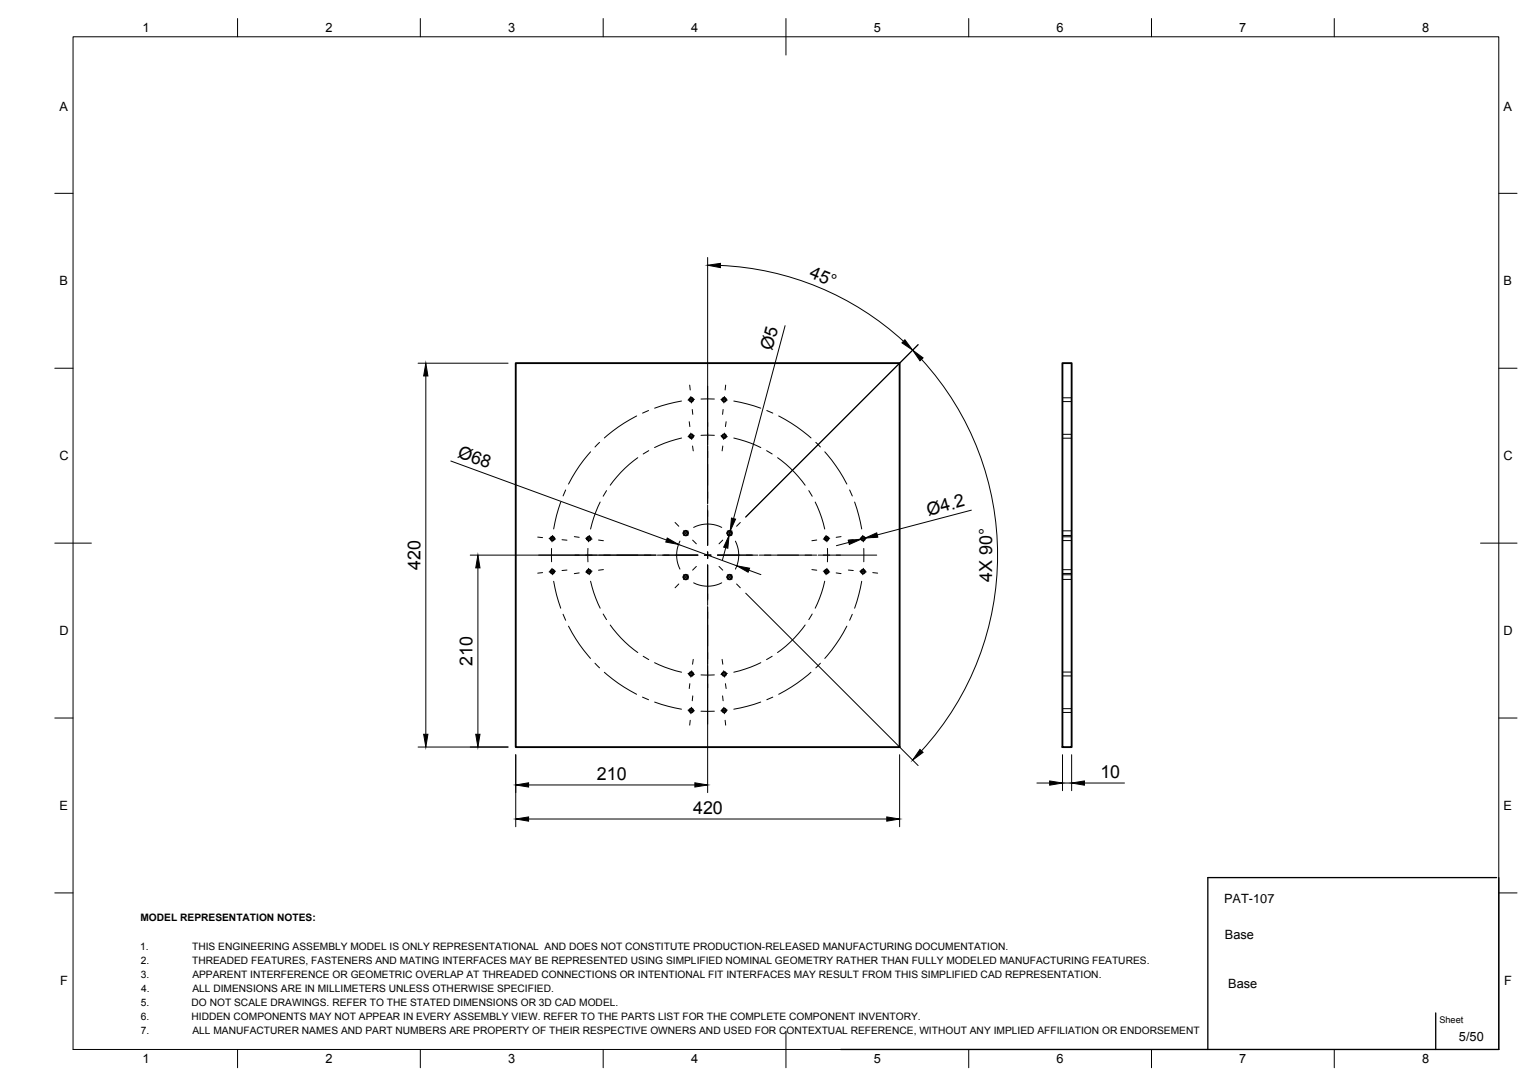
ISO-10303-21;
HEADER;
/* Generated by software containing ST-Developer
 * from STEP Tools, Inc. (www.steptools.com) 
 */

FILE_DESCRIPTION(
/* description */ ('Turntable on roller ring'),
/* implementation_level */ '2;1');

FILE_NAME(
/* name */ 'Base.step',
/* time_stamp */ '2026-10-28T03:23:59-07:00',
/* author */ (''),
/* organization */ (''),
/* preprocessor_version */ 'ST-DEVELOPER v20.2',
/* originating_system */ 'Autodesk Translation Framework v15.17.0.0',
/* authorisation */ '');

FILE_SCHEMA (('AUTOMOTIVE_DESIGN { 1 0 10303 214 3 1 1 }'));
ENDSEC;

DATA;
#10=MECHANICAL_DESIGN_GEOMETRIC_PRESENTATION_REPRESENTATION('',(#617),#16281);
#507=SHAPE_REPRESENTATION_RELATIONSHIP('SRR','None',#16521,#562);
#562=ADVANCED_BREP_SHAPE_REPRESENTATION('',(#689),#16215);
#617=STYLED_ITEM('',(#16911),#689);
#689=MANIFOLD_SOLID_BREP('Body1',#8358);
#757=FACE_BOUND('',#1780,.T.);
#758=FACE_BOUND('',#1781,.T.);
#759=FACE_BOUND('',#1782,.T.);
#760=FACE_BOUND('',#1783,.T.);
#761=FACE_BOUND('',#1784,.T.);
#762=FACE_BOUND('',#1785,.T.);
#763=FACE_BOUND('',#1786,.T.);
#764=FACE_BOUND('',#1787,.T.);
#765=FACE_BOUND('',#1788,.T.);
#766=FACE_BOUND('',#1789,.T.);
#767=FACE_BOUND('',#1790,.T.);
#768=FACE_BOUND('',#1791,.T.);
#769=FACE_BOUND('',#1792,.T.);
#770=FACE_BOUND('',#1793,.T.);
#771=FACE_BOUND('',#1794,.T.);
#772=FACE_BOUND('',#1795,.T.);
#773=FACE_BOUND('',#1796,.T.);
#774=FACE_BOUND('',#1797,.T.);
#775=FACE_BOUND('',#1798,.T.);
#776=FACE_BOUND('',#1799,.T.);
#777=FACE_BOUND('',#1801,.T.);
#778=FACE_BOUND('',#1802,.T.);
#779=FACE_BOUND('',#1803,.T.);
#780=FACE_BOUND('',#1804,.T.);
#781=FACE_BOUND('',#1805,.T.);
#782=FACE_BOUND('',#1806,.T.);
#783=FACE_BOUND('',#1807,.T.);
#784=FACE_BOUND('',#1808,.T.);
#785=FACE_BOUND('',#1809,.T.);
#786=FACE_BOUND('',#1810,.T.);
#787=FACE_BOUND('',#1811,.T.);
#788=FACE_BOUND('',#1812,.T.);
#789=FACE_BOUND('',#1813,.T.);
#790=FACE_BOUND('',#1814,.T.);
#791=FACE_BOUND('',#1815,.T.);
#792=FACE_BOUND('',#1816,.T.);
#793=FACE_BOUND('',#1817,.T.);
#794=FACE_BOUND('',#1818,.T.);
#795=FACE_BOUND('',#1819,.T.);
#796=FACE_BOUND('',#1820,.T.);
#990=PLANE('',#9103);
#991=PLANE('',#9104);
#992=PLANE('',#9105);
#993=PLANE('',#9106);
#994=PLANE('',#9107);
#995=PLANE('',#9108);
#1250=FACE_OUTER_BOUND('',#1755,.T.);
#1251=FACE_OUTER_BOUND('',#1756,.T.);
#1252=FACE_OUTER_BOUND('',#1757,.T.);
#1253=FACE_OUTER_BOUND('',#1758,.T.);
#1254=FACE_OUTER_BOUND('',#1759,.T.);
#1255=FACE_OUTER_BOUND('',#1760,.T.);
#1256=FACE_OUTER_BOUND('',#1761,.T.);
#1257=FACE_OUTER_BOUND('',#1762,.T.);
#1258=FACE_OUTER_BOUND('',#1763,.T.);
#1259=FACE_OUTER_BOUND('',#1764,.T.);
#1260=FACE_OUTER_BOUND('',#1765,.T.);
#1261=FACE_OUTER_BOUND('',#1766,.T.);
#1262=FACE_OUTER_BOUND('',#1767,.T.);
#1263=FACE_OUTER_BOUND('',#1768,.T.);
#1264=FACE_OUTER_BOUND('',#1769,.T.);
#1265=FACE_OUTER_BOUND('',#1770,.T.);
#1266=FACE_OUTER_BOUND('',#1771,.T.);
#1267=FACE_OUTER_BOUND('',#1772,.T.);
#1268=FACE_OUTER_BOUND('',#1773,.T.);
#1269=FACE_OUTER_BOUND('',#1774,.T.);
#1270=FACE_OUTER_BOUND('',#1775,.T.);
#1271=FACE_OUTER_BOUND('',#1776,.T.);
#1272=FACE_OUTER_BOUND('',#1777,.T.);
#1273=FACE_OUTER_BOUND('',#1778,.T.);
#1274=FACE_OUTER_BOUND('',#1779,.T.);
#1275=FACE_OUTER_BOUND('',#1800,.T.);
#1755=EDGE_LOOP('',(#5645,#5646,#5647,#5648));
#1756=EDGE_LOOP('',(#5649,#5650,#5651,#5652));
#1757=EDGE_LOOP('',(#5653,#5654,#5655,#5656));
#1758=EDGE_LOOP('',(#5657,#5658,#5659,#5660));
#1759=EDGE_LOOP('',(#5661,#5662,#5663,#5664));
#1760=EDGE_LOOP('',(#5665,#5666,#5667,#5668));
#1761=EDGE_LOOP('',(#5669,#5670,#5671,#5672));
#1762=EDGE_LOOP('',(#5673,#5674,#5675,#5676));
#1763=EDGE_LOOP('',(#5677,#5678,#5679,#5680));
#1764=EDGE_LOOP('',(#5681,#5682,#5683,#5684));
#1765=EDGE_LOOP('',(#5685,#5686,#5687,#5688));
#1766=EDGE_LOOP('',(#5689,#5690,#5691,#5692));
#1767=EDGE_LOOP('',(#5693,#5694,#5695,#5696));
#1768=EDGE_LOOP('',(#5697,#5698,#5699,#5700));
#1769=EDGE_LOOP('',(#5701,#5702,#5703,#5704));
#1770=EDGE_LOOP('',(#5705,#5706,#5707,#5708));
#1771=EDGE_LOOP('',(#5709,#5710,#5711,#5712));
#1772=EDGE_LOOP('',(#5713,#5714,#5715,#5716));
#1773=EDGE_LOOP('',(#5717,#5718,#5719,#5720));
#1774=EDGE_LOOP('',(#5721,#5722,#5723,#5724));
#1775=EDGE_LOOP('',(#5725,#5726,#5727,#5728));
#1776=EDGE_LOOP('',(#5729,#5730,#5731,#5732));
#1777=EDGE_LOOP('',(#5733,#5734,#5735,#5736));
#1778=EDGE_LOOP('',(#5737,#5738,#5739,#5740));
#1779=EDGE_LOOP('',(#5741,#5742,#5743,#5744));
#1780=EDGE_LOOP('',(#5745));
#1781=EDGE_LOOP('',(#5746));
#1782=EDGE_LOOP('',(#5747));
#1783=EDGE_LOOP('',(#5748));
#1784=EDGE_LOOP('',(#5749));
#1785=EDGE_LOOP('',(#5750));
#1786=EDGE_LOOP('',(#5751));
#1787=EDGE_LOOP('',(#5752));
#1788=EDGE_LOOP('',(#5753));
#1789=EDGE_LOOP('',(#5754));
#1790=EDGE_LOOP('',(#5755));
#1791=EDGE_LOOP('',(#5756));
#1792=EDGE_LOOP('',(#5757));
#1793=EDGE_LOOP('',(#5758));
#1794=EDGE_LOOP('',(#5759));
#1795=EDGE_LOOP('',(#5760));
#1796=EDGE_LOOP('',(#5761));
#1797=EDGE_LOOP('',(#5762));
#1798=EDGE_LOOP('',(#5763));
#1799=EDGE_LOOP('',(#5764));
#1800=EDGE_LOOP('',(#5765,#5766,#5767,#5768));
#1801=EDGE_LOOP('',(#5769));
#1802=EDGE_LOOP('',(#5770));
#1803=EDGE_LOOP('',(#5771));
#1804=EDGE_LOOP('',(#5772));
#1805=EDGE_LOOP('',(#5773));
#1806=EDGE_LOOP('',(#5774));
#1807=EDGE_LOOP('',(#5775));
#1808=EDGE_LOOP('',(#5776));
#1809=EDGE_LOOP('',(#5777));
#1810=EDGE_LOOP('',(#5778));
#1811=EDGE_LOOP('',(#5779));
#1812=EDGE_LOOP('',(#5780));
#1813=EDGE_LOOP('',(#5781));
#1814=EDGE_LOOP('',(#5782));
#1815=EDGE_LOOP('',(#5783));
#1816=EDGE_LOOP('',(#5784));
#1817=EDGE_LOOP('',(#5785));
#1818=EDGE_LOOP('',(#5786));
#1819=EDGE_LOOP('',(#5787));
#1820=EDGE_LOOP('',(#5788));
#2493=LINE('',#13010,#2976);
#2494=LINE('',#13016,#2977);
#2495=LINE('',#13022,#2978);
#2496=LINE('',#13028,#2979);
#2497=LINE('',#13034,#2980);
#2498=LINE('',#13040,#2981);
#2499=LINE('',#13046,#2982);
#2500=LINE('',#13052,#2983);
#2501=LINE('',#13058,#2984);
#2502=LINE('',#13064,#2985);
#2503=LINE('',#13070,#2986);
#2504=LINE('',#13076,#2987);
#2505=LINE('',#13082,#2988);
#2506=LINE('',#13088,#2989);
#2507=LINE('',#13094,#2990);
#2508=LINE('',#13100,#2991);
#2509=LINE('',#13106,#2992);
#2510=LINE('',#13112,#2993);
#2511=LINE('',#13118,#2994);
#2512=LINE('',#13124,#2995);
#2513=LINE('',#13129,#2996);
#2514=LINE('',#13131,#2997);
#2515=LINE('',#13133,#2998);
#2516=LINE('',#13134,#2999);
#2517=LINE('',#13137,#3000);
#2518=LINE('',#13139,#3001);
#2519=LINE('',#13140,#3002);
#2520=LINE('',#13143,#3003);
#2521=LINE('',#13145,#3004);
#2522=LINE('',#13146,#3005);
#2523=LINE('',#13148,#3006);
#2524=LINE('',#13149,#3007);
#2976=VECTOR('',#10210,0.210000000000001);
#2977=VECTOR('',#10217,0.210000000000001);
#2978=VECTOR('',#10224,0.210000000000001);
#2979=VECTOR('',#10231,0.210000000000001);
#2980=VECTOR('',#10238,0.21);
#2981=VECTOR('',#10245,0.21);
#2982=VECTOR('',#10252,0.21);
#2983=VECTOR('',#10259,0.21);
#2984=VECTOR('',#10266,0.210000000000001);
#2985=VECTOR('',#10273,0.210000000000001);
#2986=VECTOR('',#10280,0.210000000000001);
#2987=VECTOR('',#10287,0.210000000000001);
#2988=VECTOR('',#10294,0.21);
#2989=VECTOR('',#10301,0.21);
#2990=VECTOR('',#10308,0.21);
#2991=VECTOR('',#10315,0.21);
#2992=VECTOR('',#10322,0.25);
#2993=VECTOR('',#10329,0.25);
#2994=VECTOR('',#10336,0.25);
#2995=VECTOR('',#10343,0.25);
#2996=VECTOR('',#10348,1.);
#2997=VECTOR('',#10349,1.);
#2998=VECTOR('',#10350,1.);
#2999=VECTOR('',#10351,1.);
#3000=VECTOR('',#10354,1.);
#3001=VECTOR('',#10355,1.);
#3002=VECTOR('',#10356,1.);
#3003=VECTOR('',#10359,1.);
#3004=VECTOR('',#10360,1.);
#3005=VECTOR('',#10361,1.);
#3006=VECTOR('',#10364,1.);
#3007=VECTOR('',#10365,1.);
#3459=CIRCLE('',#9044,0.210000000000001);
#3460=CIRCLE('',#9045,0.210000000000001);
#3461=CIRCLE('',#9047,0.210000000000001);
#3462=CIRCLE('',#9048,0.210000000000001);
#3463=CIRCLE('',#9050,0.210000000000001);
#3464=CIRCLE('',#9051,0.210000000000001);
#3465=CIRCLE('',#9053,0.210000000000001);
#3466=CIRCLE('',#9054,0.210000000000001);
#3467=CIRCLE('',#9056,0.21);
#3468=CIRCLE('',#9057,0.21);
#3469=CIRCLE('',#9059,0.21);
#3470=CIRCLE('',#9060,0.21);
#3471=CIRCLE('',#9062,0.21);
#3472=CIRCLE('',#9063,0.21);
#3473=CIRCLE('',#9065,0.21);
#3474=CIRCLE('',#9066,0.21);
#3475=CIRCLE('',#9068,0.210000000000001);
#3476=CIRCLE('',#9069,0.210000000000001);
#3477=CIRCLE('',#9071,0.210000000000001);
#3478=CIRCLE('',#9072,0.210000000000001);
#3479=CIRCLE('',#9074,0.210000000000001);
#3480=CIRCLE('',#9075,0.210000000000001);
#3481=CIRCLE('',#9077,0.210000000000001);
#3482=CIRCLE('',#9078,0.210000000000001);
#3483=CIRCLE('',#9080,0.21);
#3484=CIRCLE('',#9081,0.21);
#3485=CIRCLE('',#9083,0.21);
#3486=CIRCLE('',#9084,0.21);
#3487=CIRCLE('',#9086,0.21);
#3488=CIRCLE('',#9087,0.21);
#3489=CIRCLE('',#9089,0.21);
#3490=CIRCLE('',#9090,0.21);
#3491=CIRCLE('',#9092,0.25);
#3492=CIRCLE('',#9093,0.25);
#3493=CIRCLE('',#9095,0.25);
#3494=CIRCLE('',#9096,0.25);
#3495=CIRCLE('',#9098,0.25);
#3496=CIRCLE('',#9099,0.25);
#3497=CIRCLE('',#9101,0.25);
#3498=CIRCLE('',#9102,0.25);
#3949=VERTEX_POINT('',#13007);
#3950=VERTEX_POINT('',#13009);
#3951=VERTEX_POINT('',#13013);
#3952=VERTEX_POINT('',#13015);
#3953=VERTEX_POINT('',#13019);
#3954=VERTEX_POINT('',#13021);
#3955=VERTEX_POINT('',#13025);
#3956=VERTEX_POINT('',#13027);
#3957=VERTEX_POINT('',#13031);
#3958=VERTEX_POINT('',#13033);
#3959=VERTEX_POINT('',#13037);
#3960=VERTEX_POINT('',#13039);
#3961=VERTEX_POINT('',#13043);
#3962=VERTEX_POINT('',#13045);
#3963=VERTEX_POINT('',#13049);
#3964=VERTEX_POINT('',#13051);
#3965=VERTEX_POINT('',#13055);
#3966=VERTEX_POINT('',#13057);
#3967=VERTEX_POINT('',#13061);
#3968=VERTEX_POINT('',#13063);
#3969=VERTEX_POINT('',#13067);
#3970=VERTEX_POINT('',#13069);
#3971=VERTEX_POINT('',#13073);
#3972=VERTEX_POINT('',#13075);
#3973=VERTEX_POINT('',#13079);
#3974=VERTEX_POINT('',#13081);
#3975=VERTEX_POINT('',#13085);
#3976=VERTEX_POINT('',#13087);
#3977=VERTEX_POINT('',#13091);
#3978=VERTEX_POINT('',#13093);
#3979=VERTEX_POINT('',#13097);
#3980=VERTEX_POINT('',#13099);
#3981=VERTEX_POINT('',#13103);
#3982=VERTEX_POINT('',#13105);
#3983=VERTEX_POINT('',#13109);
#3984=VERTEX_POINT('',#13111);
#3985=VERTEX_POINT('',#13115);
#3986=VERTEX_POINT('',#13117);
#3987=VERTEX_POINT('',#13121);
#3988=VERTEX_POINT('',#13123);
#3989=VERTEX_POINT('',#13127);
#3990=VERTEX_POINT('',#13128);
#3991=VERTEX_POINT('',#13130);
#3992=VERTEX_POINT('',#13132);
#3993=VERTEX_POINT('',#13136);
#3994=VERTEX_POINT('',#13138);
#3995=VERTEX_POINT('',#13142);
#3996=VERTEX_POINT('',#13144);
#4633=EDGE_CURVE('',#3949,#3949,#3459,.T.);
#4634=EDGE_CURVE('',#3949,#3950,#2493,.T.);
#4635=EDGE_CURVE('',#3950,#3950,#3460,.T.);
#4636=EDGE_CURVE('',#3951,#3951,#3461,.T.);
#4637=EDGE_CURVE('',#3951,#3952,#2494,.T.);
#4638=EDGE_CURVE('',#3952,#3952,#3462,.T.);
#4639=EDGE_CURVE('',#3953,#3953,#3463,.T.);
#4640=EDGE_CURVE('',#3953,#3954,#2495,.T.);
#4641=EDGE_CURVE('',#3954,#3954,#3464,.T.);
#4642=EDGE_CURVE('',#3955,#3955,#3465,.T.);
#4643=EDGE_CURVE('',#3955,#3956,#2496,.T.);
#4644=EDGE_CURVE('',#3956,#3956,#3466,.T.);
#4645=EDGE_CURVE('',#3957,#3957,#3467,.T.);
#4646=EDGE_CURVE('',#3957,#3958,#2497,.T.);
#4647=EDGE_CURVE('',#3958,#3958,#3468,.T.);
#4648=EDGE_CURVE('',#3959,#3959,#3469,.T.);
#4649=EDGE_CURVE('',#3959,#3960,#2498,.T.);
#4650=EDGE_CURVE('',#3960,#3960,#3470,.T.);
#4651=EDGE_CURVE('',#3961,#3961,#3471,.T.);
#4652=EDGE_CURVE('',#3961,#3962,#2499,.T.);
#4653=EDGE_CURVE('',#3962,#3962,#3472,.T.);
#4654=EDGE_CURVE('',#3963,#3963,#3473,.T.);
#4655=EDGE_CURVE('',#3963,#3964,#2500,.T.);
#4656=EDGE_CURVE('',#3964,#3964,#3474,.T.);
#4657=EDGE_CURVE('',#3965,#3965,#3475,.T.);
#4658=EDGE_CURVE('',#3965,#3966,#2501,.T.);
#4659=EDGE_CURVE('',#3966,#3966,#3476,.T.);
#4660=EDGE_CURVE('',#3967,#3967,#3477,.T.);
#4661=EDGE_CURVE('',#3967,#3968,#2502,.T.);
#4662=EDGE_CURVE('',#3968,#3968,#3478,.T.);
#4663=EDGE_CURVE('',#3969,#3969,#3479,.T.);
#4664=EDGE_CURVE('',#3969,#3970,#2503,.T.);
#4665=EDGE_CURVE('',#3970,#3970,#3480,.T.);
#4666=EDGE_CURVE('',#3971,#3971,#3481,.T.);
#4667=EDGE_CURVE('',#3971,#3972,#2504,.T.);
#4668=EDGE_CURVE('',#3972,#3972,#3482,.T.);
#4669=EDGE_CURVE('',#3973,#3973,#3483,.T.);
#4670=EDGE_CURVE('',#3973,#3974,#2505,.T.);
#4671=EDGE_CURVE('',#3974,#3974,#3484,.T.);
#4672=EDGE_CURVE('',#3975,#3975,#3485,.T.);
#4673=EDGE_CURVE('',#3975,#3976,#2506,.T.);
#4674=EDGE_CURVE('',#3976,#3976,#3486,.T.);
#4675=EDGE_CURVE('',#3977,#3977,#3487,.T.);
#4676=EDGE_CURVE('',#3977,#3978,#2507,.T.);
#4677=EDGE_CURVE('',#3978,#3978,#3488,.T.);
#4678=EDGE_CURVE('',#3979,#3979,#3489,.T.);
#4679=EDGE_CURVE('',#3979,#3980,#2508,.T.);
#4680=EDGE_CURVE('',#3980,#3980,#3490,.T.);
#4681=EDGE_CURVE('',#3981,#3981,#3491,.T.);
#4682=EDGE_CURVE('',#3981,#3982,#2509,.T.);
#4683=EDGE_CURVE('',#3982,#3982,#3492,.T.);
#4684=EDGE_CURVE('',#3983,#3983,#3493,.T.);
#4685=EDGE_CURVE('',#3983,#3984,#2510,.T.);
#4686=EDGE_CURVE('',#3984,#3984,#3494,.T.);
#4687=EDGE_CURVE('',#3985,#3985,#3495,.T.);
#4688=EDGE_CURVE('',#3985,#3986,#2511,.T.);
#4689=EDGE_CURVE('',#3986,#3986,#3496,.T.);
#4690=EDGE_CURVE('',#3987,#3987,#3497,.T.);
#4691=EDGE_CURVE('',#3987,#3988,#2512,.T.);
#4692=EDGE_CURVE('',#3988,#3988,#3498,.T.);
#4693=EDGE_CURVE('',#3989,#3990,#2513,.T.);
#4694=EDGE_CURVE('',#3990,#3991,#2514,.T.);
#4695=EDGE_CURVE('',#3992,#3991,#2515,.T.);
#4696=EDGE_CURVE('',#3989,#3992,#2516,.T.);
#4697=EDGE_CURVE('',#3993,#3989,#2517,.T.);
#4698=EDGE_CURVE('',#3994,#3992,#2518,.T.);
#4699=EDGE_CURVE('',#3993,#3994,#2519,.T.);
#4700=EDGE_CURVE('',#3995,#3993,#2520,.T.);
#4701=EDGE_CURVE('',#3996,#3994,#2521,.T.);
#4702=EDGE_CURVE('',#3995,#3996,#2522,.T.);
#4703=EDGE_CURVE('',#3990,#3995,#2523,.T.);
#4704=EDGE_CURVE('',#3991,#3996,#2524,.T.);
#5645=ORIENTED_EDGE('',*,*,#4633,.F.);
#5646=ORIENTED_EDGE('',*,*,#4634,.T.);
#5647=ORIENTED_EDGE('',*,*,#4635,.F.);
#5648=ORIENTED_EDGE('',*,*,#4634,.F.);
#5649=ORIENTED_EDGE('',*,*,#4636,.F.);
#5650=ORIENTED_EDGE('',*,*,#4637,.T.);
#5651=ORIENTED_EDGE('',*,*,#4638,.F.);
#5652=ORIENTED_EDGE('',*,*,#4637,.F.);
#5653=ORIENTED_EDGE('',*,*,#4639,.F.);
#5654=ORIENTED_EDGE('',*,*,#4640,.T.);
#5655=ORIENTED_EDGE('',*,*,#4641,.F.);
#5656=ORIENTED_EDGE('',*,*,#4640,.F.);
#5657=ORIENTED_EDGE('',*,*,#4642,.F.);
#5658=ORIENTED_EDGE('',*,*,#4643,.T.);
#5659=ORIENTED_EDGE('',*,*,#4644,.F.);
#5660=ORIENTED_EDGE('',*,*,#4643,.F.);
#5661=ORIENTED_EDGE('',*,*,#4645,.F.);
#5662=ORIENTED_EDGE('',*,*,#4646,.T.);
#5663=ORIENTED_EDGE('',*,*,#4647,.F.);
#5664=ORIENTED_EDGE('',*,*,#4646,.F.);
#5665=ORIENTED_EDGE('',*,*,#4648,.F.);
#5666=ORIENTED_EDGE('',*,*,#4649,.T.);
#5667=ORIENTED_EDGE('',*,*,#4650,.F.);
#5668=ORIENTED_EDGE('',*,*,#4649,.F.);
#5669=ORIENTED_EDGE('',*,*,#4651,.F.);
#5670=ORIENTED_EDGE('',*,*,#4652,.T.);
#5671=ORIENTED_EDGE('',*,*,#4653,.F.);
#5672=ORIENTED_EDGE('',*,*,#4652,.F.);
#5673=ORIENTED_EDGE('',*,*,#4654,.F.);
#5674=ORIENTED_EDGE('',*,*,#4655,.T.);
#5675=ORIENTED_EDGE('',*,*,#4656,.F.);
#5676=ORIENTED_EDGE('',*,*,#4655,.F.);
#5677=ORIENTED_EDGE('',*,*,#4657,.F.);
#5678=ORIENTED_EDGE('',*,*,#4658,.T.);
#5679=ORIENTED_EDGE('',*,*,#4659,.F.);
#5680=ORIENTED_EDGE('',*,*,#4658,.F.);
#5681=ORIENTED_EDGE('',*,*,#4660,.F.);
#5682=ORIENTED_EDGE('',*,*,#4661,.T.);
#5683=ORIENTED_EDGE('',*,*,#4662,.F.);
#5684=ORIENTED_EDGE('',*,*,#4661,.F.);
#5685=ORIENTED_EDGE('',*,*,#4663,.F.);
#5686=ORIENTED_EDGE('',*,*,#4664,.T.);
#5687=ORIENTED_EDGE('',*,*,#4665,.F.);
#5688=ORIENTED_EDGE('',*,*,#4664,.F.);
#5689=ORIENTED_EDGE('',*,*,#4666,.F.);
#5690=ORIENTED_EDGE('',*,*,#4667,.T.);
#5691=ORIENTED_EDGE('',*,*,#4668,.F.);
#5692=ORIENTED_EDGE('',*,*,#4667,.F.);
#5693=ORIENTED_EDGE('',*,*,#4669,.F.);
#5694=ORIENTED_EDGE('',*,*,#4670,.T.);
#5695=ORIENTED_EDGE('',*,*,#4671,.F.);
#5696=ORIENTED_EDGE('',*,*,#4670,.F.);
#5697=ORIENTED_EDGE('',*,*,#4672,.F.);
#5698=ORIENTED_EDGE('',*,*,#4673,.T.);
#5699=ORIENTED_EDGE('',*,*,#4674,.F.);
#5700=ORIENTED_EDGE('',*,*,#4673,.F.);
#5701=ORIENTED_EDGE('',*,*,#4675,.F.);
#5702=ORIENTED_EDGE('',*,*,#4676,.T.);
#5703=ORIENTED_EDGE('',*,*,#4677,.F.);
#5704=ORIENTED_EDGE('',*,*,#4676,.F.);
#5705=ORIENTED_EDGE('',*,*,#4678,.F.);
#5706=ORIENTED_EDGE('',*,*,#4679,.T.);
#5707=ORIENTED_EDGE('',*,*,#4680,.F.);
#5708=ORIENTED_EDGE('',*,*,#4679,.F.);
#5709=ORIENTED_EDGE('',*,*,#4681,.F.);
#5710=ORIENTED_EDGE('',*,*,#4682,.T.);
#5711=ORIENTED_EDGE('',*,*,#4683,.F.);
#5712=ORIENTED_EDGE('',*,*,#4682,.F.);
#5713=ORIENTED_EDGE('',*,*,#4684,.F.);
#5714=ORIENTED_EDGE('',*,*,#4685,.T.);
#5715=ORIENTED_EDGE('',*,*,#4686,.F.);
#5716=ORIENTED_EDGE('',*,*,#4685,.F.);
#5717=ORIENTED_EDGE('',*,*,#4687,.F.);
#5718=ORIENTED_EDGE('',*,*,#4688,.T.);
#5719=ORIENTED_EDGE('',*,*,#4689,.F.);
#5720=ORIENTED_EDGE('',*,*,#4688,.F.);
#5721=ORIENTED_EDGE('',*,*,#4690,.F.);
#5722=ORIENTED_EDGE('',*,*,#4691,.T.);
#5723=ORIENTED_EDGE('',*,*,#4692,.F.);
#5724=ORIENTED_EDGE('',*,*,#4691,.F.);
#5725=ORIENTED_EDGE('',*,*,#4693,.T.);
#5726=ORIENTED_EDGE('',*,*,#4694,.T.);
#5727=ORIENTED_EDGE('',*,*,#4695,.F.);
#5728=ORIENTED_EDGE('',*,*,#4696,.F.);
#5729=ORIENTED_EDGE('',*,*,#4697,.T.);
#5730=ORIENTED_EDGE('',*,*,#4696,.T.);
#5731=ORIENTED_EDGE('',*,*,#4698,.F.);
#5732=ORIENTED_EDGE('',*,*,#4699,.F.);
#5733=ORIENTED_EDGE('',*,*,#4700,.T.);
#5734=ORIENTED_EDGE('',*,*,#4699,.T.);
#5735=ORIENTED_EDGE('',*,*,#4701,.F.);
#5736=ORIENTED_EDGE('',*,*,#4702,.F.);
#5737=ORIENTED_EDGE('',*,*,#4703,.T.);
#5738=ORIENTED_EDGE('',*,*,#4702,.T.);
#5739=ORIENTED_EDGE('',*,*,#4704,.F.);
#5740=ORIENTED_EDGE('',*,*,#4694,.F.);
#5741=ORIENTED_EDGE('',*,*,#4704,.T.);
#5742=ORIENTED_EDGE('',*,*,#4701,.T.);
#5743=ORIENTED_EDGE('',*,*,#4698,.T.);
#5744=ORIENTED_EDGE('',*,*,#4695,.T.);
#5745=ORIENTED_EDGE('',*,*,#4647,.T.);
#5746=ORIENTED_EDGE('',*,*,#4650,.T.);
#5747=ORIENTED_EDGE('',*,*,#4653,.T.);
#5748=ORIENTED_EDGE('',*,*,#4656,.T.);
#5749=ORIENTED_EDGE('',*,*,#4671,.T.);
#5750=ORIENTED_EDGE('',*,*,#4674,.T.);
#5751=ORIENTED_EDGE('',*,*,#4677,.T.);
#5752=ORIENTED_EDGE('',*,*,#4680,.T.);
#5753=ORIENTED_EDGE('',*,*,#4683,.T.);
#5754=ORIENTED_EDGE('',*,*,#4686,.T.);
#5755=ORIENTED_EDGE('',*,*,#4689,.T.);
#5756=ORIENTED_EDGE('',*,*,#4692,.T.);
#5757=ORIENTED_EDGE('',*,*,#4668,.T.);
#5758=ORIENTED_EDGE('',*,*,#4665,.T.);
#5759=ORIENTED_EDGE('',*,*,#4662,.T.);
#5760=ORIENTED_EDGE('',*,*,#4659,.T.);
#5761=ORIENTED_EDGE('',*,*,#4644,.T.);
#5762=ORIENTED_EDGE('',*,*,#4641,.T.);
#5763=ORIENTED_EDGE('',*,*,#4638,.T.);
#5764=ORIENTED_EDGE('',*,*,#4635,.T.);
#5765=ORIENTED_EDGE('',*,*,#4703,.F.);
#5766=ORIENTED_EDGE('',*,*,#4693,.F.);
#5767=ORIENTED_EDGE('',*,*,#4697,.F.);
#5768=ORIENTED_EDGE('',*,*,#4700,.F.);
#5769=ORIENTED_EDGE('',*,*,#4645,.T.);
#5770=ORIENTED_EDGE('',*,*,#4648,.T.);
#5771=ORIENTED_EDGE('',*,*,#4651,.T.);
#5772=ORIENTED_EDGE('',*,*,#4654,.T.);
#5773=ORIENTED_EDGE('',*,*,#4669,.T.);
#5774=ORIENTED_EDGE('',*,*,#4672,.T.);
#5775=ORIENTED_EDGE('',*,*,#4675,.T.);
#5776=ORIENTED_EDGE('',*,*,#4678,.T.);
#5777=ORIENTED_EDGE('',*,*,#4681,.T.);
#5778=ORIENTED_EDGE('',*,*,#4684,.T.);
#5779=ORIENTED_EDGE('',*,*,#4687,.T.);
#5780=ORIENTED_EDGE('',*,*,#4690,.T.);
#5781=ORIENTED_EDGE('',*,*,#4666,.T.);
#5782=ORIENTED_EDGE('',*,*,#4663,.T.);
#5783=ORIENTED_EDGE('',*,*,#4660,.T.);
#5784=ORIENTED_EDGE('',*,*,#4657,.T.);
#5785=ORIENTED_EDGE('',*,*,#4642,.T.);
#5786=ORIENTED_EDGE('',*,*,#4639,.T.);
#5787=ORIENTED_EDGE('',*,*,#4636,.T.);
#5788=ORIENTED_EDGE('',*,*,#4633,.T.);
#7669=CYLINDRICAL_SURFACE('',#9043,0.210000000000001);
#7670=CYLINDRICAL_SURFACE('',#9046,0.210000000000001);
#7671=CYLINDRICAL_SURFACE('',#9049,0.210000000000001);
#7672=CYLINDRICAL_SURFACE('',#9052,0.210000000000001);
#7673=CYLINDRICAL_SURFACE('',#9055,0.21);
#7674=CYLINDRICAL_SURFACE('',#9058,0.21);
#7675=CYLINDRICAL_SURFACE('',#9061,0.21);
#7676=CYLINDRICAL_SURFACE('',#9064,0.21);
#7677=CYLINDRICAL_SURFACE('',#9067,0.210000000000001);
#7678=CYLINDRICAL_SURFACE('',#9070,0.210000000000001);
#7679=CYLINDRICAL_SURFACE('',#9073,0.210000000000001);
#7680=CYLINDRICAL_SURFACE('',#9076,0.210000000000001);
#7681=CYLINDRICAL_SURFACE('',#9079,0.21);
#7682=CYLINDRICAL_SURFACE('',#9082,0.21);
#7683=CYLINDRICAL_SURFACE('',#9085,0.21);
#7684=CYLINDRICAL_SURFACE('',#9088,0.21);
#7685=CYLINDRICAL_SURFACE('',#9091,0.25);
#7686=CYLINDRICAL_SURFACE('',#9094,0.25);
#7687=CYLINDRICAL_SURFACE('',#9097,0.25);
#7688=CYLINDRICAL_SURFACE('',#9100,0.25);
#7853=ADVANCED_FACE('',(#1250),#7669,.F.);
#7854=ADVANCED_FACE('',(#1251),#7670,.F.);
#7855=ADVANCED_FACE('',(#1252),#7671,.F.);
#7856=ADVANCED_FACE('',(#1253),#7672,.F.);
#7857=ADVANCED_FACE('',(#1254),#7673,.F.);
#7858=ADVANCED_FACE('',(#1255),#7674,.F.);
#7859=ADVANCED_FACE('',(#1256),#7675,.F.);
#7860=ADVANCED_FACE('',(#1257),#7676,.F.);
#7861=ADVANCED_FACE('',(#1258),#7677,.F.);
#7862=ADVANCED_FACE('',(#1259),#7678,.F.);
#7863=ADVANCED_FACE('',(#1260),#7679,.F.);
#7864=ADVANCED_FACE('',(#1261),#7680,.F.);
#7865=ADVANCED_FACE('',(#1262),#7681,.F.);
#7866=ADVANCED_FACE('',(#1263),#7682,.F.);
#7867=ADVANCED_FACE('',(#1264),#7683,.F.);
#7868=ADVANCED_FACE('',(#1265),#7684,.F.);
#7869=ADVANCED_FACE('',(#1266),#7685,.F.);
#7870=ADVANCED_FACE('',(#1267),#7686,.F.);
#7871=ADVANCED_FACE('',(#1268),#7687,.F.);
#7872=ADVANCED_FACE('',(#1269),#7688,.F.);
#7873=ADVANCED_FACE('',(#1270),#990,.T.);
#7874=ADVANCED_FACE('',(#1271),#991,.T.);
#7875=ADVANCED_FACE('',(#1272),#992,.T.);
#7876=ADVANCED_FACE('',(#1273),#993,.T.);
#7877=ADVANCED_FACE('',(#1274,#757,#758,#759,#760,#761,#762,#763,#764,#765,
#766,#767,#768,#769,#770,#771,#772,#773,#774,#775,#776),#994,.T.);
#7878=ADVANCED_FACE('',(#1275,#777,#778,#779,#780,#781,#782,#783,#784,#785,
#786,#787,#788,#789,#790,#791,#792,#793,#794,#795,#796),#995,.F.);
#8358=CLOSED_SHELL('',(#7853,#7854,#7855,#7856,#7857,#7858,#7859,#7860,
#7861,#7862,#7863,#7864,#7865,#7866,#7867,#7868,#7869,#7870,#7871,#7872,
#7873,#7874,#7875,#7876,#7877,#7878));
#9042=AXIS2_PLACEMENT_3D('',#13005,#10204,#10205);
#9043=AXIS2_PLACEMENT_3D('',#13006,#10206,#10207);
#9044=AXIS2_PLACEMENT_3D('',#13008,#10208,#10209);
#9045=AXIS2_PLACEMENT_3D('',#13011,#10211,#10212);
#9046=AXIS2_PLACEMENT_3D('',#13012,#10213,#10214);
#9047=AXIS2_PLACEMENT_3D('',#13014,#10215,#10216);
#9048=AXIS2_PLACEMENT_3D('',#13017,#10218,#10219);
#9049=AXIS2_PLACEMENT_3D('',#13018,#10220,#10221);
#9050=AXIS2_PLACEMENT_3D('',#13020,#10222,#10223);
#9051=AXIS2_PLACEMENT_3D('',#13023,#10225,#10226);
#9052=AXIS2_PLACEMENT_3D('',#13024,#10227,#10228);
#9053=AXIS2_PLACEMENT_3D('',#13026,#10229,#10230);
#9054=AXIS2_PLACEMENT_3D('',#13029,#10232,#10233);
#9055=AXIS2_PLACEMENT_3D('',#13030,#10234,#10235);
#9056=AXIS2_PLACEMENT_3D('',#13032,#10236,#10237);
#9057=AXIS2_PLACEMENT_3D('',#13035,#10239,#10240);
#9058=AXIS2_PLACEMENT_3D('',#13036,#10241,#10242);
#9059=AXIS2_PLACEMENT_3D('',#13038,#10243,#10244);
#9060=AXIS2_PLACEMENT_3D('',#13041,#10246,#10247);
#9061=AXIS2_PLACEMENT_3D('',#13042,#10248,#10249);
#9062=AXIS2_PLACEMENT_3D('',#13044,#10250,#10251);
#9063=AXIS2_PLACEMENT_3D('',#13047,#10253,#10254);
#9064=AXIS2_PLACEMENT_3D('',#13048,#10255,#10256);
#9065=AXIS2_PLACEMENT_3D('',#13050,#10257,#10258);
#9066=AXIS2_PLACEMENT_3D('',#13053,#10260,#10261);
#9067=AXIS2_PLACEMENT_3D('',#13054,#10262,#10263);
#9068=AXIS2_PLACEMENT_3D('',#13056,#10264,#10265);
#9069=AXIS2_PLACEMENT_3D('',#13059,#10267,#10268);
#9070=AXIS2_PLACEMENT_3D('',#13060,#10269,#10270);
#9071=AXIS2_PLACEMENT_3D('',#13062,#10271,#10272);
#9072=AXIS2_PLACEMENT_3D('',#13065,#10274,#10275);
#9073=AXIS2_PLACEMENT_3D('',#13066,#10276,#10277);
#9074=AXIS2_PLACEMENT_3D('',#13068,#10278,#10279);
#9075=AXIS2_PLACEMENT_3D('',#13071,#10281,#10282);
#9076=AXIS2_PLACEMENT_3D('',#13072,#10283,#10284);
#9077=AXIS2_PLACEMENT_3D('',#13074,#10285,#10286);
#9078=AXIS2_PLACEMENT_3D('',#13077,#10288,#10289);
#9079=AXIS2_PLACEMENT_3D('',#13078,#10290,#10291);
#9080=AXIS2_PLACEMENT_3D('',#13080,#10292,#10293);
#9081=AXIS2_PLACEMENT_3D('',#13083,#10295,#10296);
#9082=AXIS2_PLACEMENT_3D('',#13084,#10297,#10298);
#9083=AXIS2_PLACEMENT_3D('',#13086,#10299,#10300);
#9084=AXIS2_PLACEMENT_3D('',#13089,#10302,#10303);
#9085=AXIS2_PLACEMENT_3D('',#13090,#10304,#10305);
#9086=AXIS2_PLACEMENT_3D('',#13092,#10306,#10307);
#9087=AXIS2_PLACEMENT_3D('',#13095,#10309,#10310);
#9088=AXIS2_PLACEMENT_3D('',#13096,#10311,#10312);
#9089=AXIS2_PLACEMENT_3D('',#13098,#10313,#10314);
#9090=AXIS2_PLACEMENT_3D('',#13101,#10316,#10317);
#9091=AXIS2_PLACEMENT_3D('',#13102,#10318,#10319);
#9092=AXIS2_PLACEMENT_3D('',#13104,#10320,#10321);
#9093=AXIS2_PLACEMENT_3D('',#13107,#10323,#10324);
#9094=AXIS2_PLACEMENT_3D('',#13108,#10325,#10326);
#9095=AXIS2_PLACEMENT_3D('',#13110,#10327,#10328);
#9096=AXIS2_PLACEMENT_3D('',#13113,#10330,#10331);
#9097=AXIS2_PLACEMENT_3D('',#13114,#10332,#10333);
#9098=AXIS2_PLACEMENT_3D('',#13116,#10334,#10335);
#9099=AXIS2_PLACEMENT_3D('',#13119,#10337,#10338);
#9100=AXIS2_PLACEMENT_3D('',#13120,#10339,#10340);
#9101=AXIS2_PLACEMENT_3D('',#13122,#10341,#10342);
#9102=AXIS2_PLACEMENT_3D('',#13125,#10344,#10345);
#9103=AXIS2_PLACEMENT_3D('',#13126,#10346,#10347);
#9104=AXIS2_PLACEMENT_3D('',#13135,#10352,#10353);
#9105=AXIS2_PLACEMENT_3D('',#13141,#10357,#10358);
#9106=AXIS2_PLACEMENT_3D('',#13147,#10362,#10363);
#9107=AXIS2_PLACEMENT_3D('',#13150,#10366,#10367);
#9108=AXIS2_PLACEMENT_3D('',#13151,#10368,#10369);
#10204=DIRECTION('axis',(0.,0.,1.));
#10205=DIRECTION('refdir',(1.,0.,0.));
#10206=DIRECTION('center_axis',(0.,0.,1.));
#10207=DIRECTION('ref_axis',(1.,0.,0.));
#10208=DIRECTION('center_axis',(0.,0.,1.));
#10209=DIRECTION('ref_axis',(1.,0.,0.));
#10210=DIRECTION('',(0.,0.,1.));
#10211=DIRECTION('center_axis',(0.,0.,-1.));
#10212=DIRECTION('ref_axis',(1.,0.,0.));
#10213=DIRECTION('center_axis',(0.,0.,1.));
#10214=DIRECTION('ref_axis',(1.,0.,0.));
#10215=DIRECTION('center_axis',(0.,0.,1.));
#10216=DIRECTION('ref_axis',(1.,0.,0.));
#10217=DIRECTION('',(0.,0.,1.));
#10218=DIRECTION('center_axis',(0.,0.,-1.));
#10219=DIRECTION('ref_axis',(1.,0.,0.));
#10220=DIRECTION('center_axis',(0.,0.,1.));
#10221=DIRECTION('ref_axis',(1.,0.,0.));
#10222=DIRECTION('center_axis',(0.,0.,1.));
#10223=DIRECTION('ref_axis',(1.,0.,0.));
#10224=DIRECTION('',(0.,0.,1.));
#10225=DIRECTION('center_axis',(0.,0.,-1.));
#10226=DIRECTION('ref_axis',(1.,0.,0.));
#10227=DIRECTION('center_axis',(0.,0.,1.));
#10228=DIRECTION('ref_axis',(1.,0.,0.));
#10229=DIRECTION('center_axis',(0.,0.,1.));
#10230=DIRECTION('ref_axis',(1.,0.,0.));
#10231=DIRECTION('',(0.,0.,1.));
#10232=DIRECTION('center_axis',(0.,0.,-1.));
#10233=DIRECTION('ref_axis',(1.,0.,0.));
#10234=DIRECTION('center_axis',(0.,0.,1.));
#10235=DIRECTION('ref_axis',(1.,0.,0.));
#10236=DIRECTION('center_axis',(0.,0.,1.));
#10237=DIRECTION('ref_axis',(1.,0.,0.));
#10238=DIRECTION('',(0.,0.,1.));
#10239=DIRECTION('center_axis',(0.,0.,-1.));
#10240=DIRECTION('ref_axis',(1.,0.,0.));
#10241=DIRECTION('center_axis',(0.,0.,1.));
#10242=DIRECTION('ref_axis',(1.,0.,0.));
#10243=DIRECTION('center_axis',(0.,0.,1.));
#10244=DIRECTION('ref_axis',(1.,0.,0.));
#10245=DIRECTION('',(0.,0.,1.));
#10246=DIRECTION('center_axis',(0.,0.,-1.));
#10247=DIRECTION('ref_axis',(1.,0.,0.));
#10248=DIRECTION('center_axis',(0.,0.,1.));
#10249=DIRECTION('ref_axis',(1.,0.,0.));
#10250=DIRECTION('center_axis',(0.,0.,1.));
#10251=DIRECTION('ref_axis',(1.,0.,0.));
#10252=DIRECTION('',(0.,0.,1.));
#10253=DIRECTION('center_axis',(0.,0.,-1.));
#10254=DIRECTION('ref_axis',(1.,0.,0.));
#10255=DIRECTION('center_axis',(0.,0.,1.));
#10256=DIRECTION('ref_axis',(1.,0.,0.));
#10257=DIRECTION('center_axis',(0.,0.,1.));
#10258=DIRECTION('ref_axis',(1.,0.,0.));
#10259=DIRECTION('',(0.,0.,1.));
#10260=DIRECTION('center_axis',(0.,0.,-1.));
#10261=DIRECTION('ref_axis',(1.,0.,0.));
#10262=DIRECTION('center_axis',(0.,0.,1.));
#10263=DIRECTION('ref_axis',(1.,0.,0.));
#10264=DIRECTION('center_axis',(0.,0.,1.));
#10265=DIRECTION('ref_axis',(1.,0.,0.));
#10266=DIRECTION('',(0.,0.,1.));
#10267=DIRECTION('center_axis',(0.,0.,-1.));
#10268=DIRECTION('ref_axis',(1.,0.,0.));
#10269=DIRECTION('center_axis',(0.,0.,1.));
#10270=DIRECTION('ref_axis',(1.,0.,0.));
#10271=DIRECTION('center_axis',(0.,0.,1.));
#10272=DIRECTION('ref_axis',(1.,0.,0.));
#10273=DIRECTION('',(0.,0.,1.));
#10274=DIRECTION('center_axis',(0.,0.,-1.));
#10275=DIRECTION('ref_axis',(1.,0.,0.));
#10276=DIRECTION('center_axis',(0.,0.,1.));
#10277=DIRECTION('ref_axis',(1.,0.,0.));
#10278=DIRECTION('center_axis',(0.,0.,1.));
#10279=DIRECTION('ref_axis',(1.,0.,0.));
#10280=DIRECTION('',(0.,0.,1.));
#10281=DIRECTION('center_axis',(0.,0.,-1.));
#10282=DIRECTION('ref_axis',(1.,0.,0.));
#10283=DIRECTION('center_axis',(0.,0.,1.));
#10284=DIRECTION('ref_axis',(1.,0.,0.));
#10285=DIRECTION('center_axis',(0.,0.,1.));
#10286=DIRECTION('ref_axis',(1.,0.,0.));
#10287=DIRECTION('',(0.,0.,1.));
#10288=DIRECTION('center_axis',(0.,0.,-1.));
#10289=DIRECTION('ref_axis',(1.,0.,0.));
#10290=DIRECTION('center_axis',(0.,0.,1.));
#10291=DIRECTION('ref_axis',(1.,0.,0.));
#10292=DIRECTION('center_axis',(0.,0.,1.));
#10293=DIRECTION('ref_axis',(1.,0.,0.));
#10294=DIRECTION('',(0.,0.,1.));
#10295=DIRECTION('center_axis',(0.,0.,-1.));
#10296=DIRECTION('ref_axis',(1.,0.,0.));
#10297=DIRECTION('center_axis',(0.,0.,1.));
#10298=DIRECTION('ref_axis',(1.,0.,0.));
#10299=DIRECTION('center_axis',(0.,0.,1.));
#10300=DIRECTION('ref_axis',(1.,0.,0.));
#10301=DIRECTION('',(0.,0.,1.));
#10302=DIRECTION('center_axis',(0.,0.,-1.));
#10303=DIRECTION('ref_axis',(1.,0.,0.));
#10304=DIRECTION('center_axis',(0.,0.,1.));
#10305=DIRECTION('ref_axis',(1.,0.,0.));
#10306=DIRECTION('center_axis',(0.,0.,1.));
#10307=DIRECTION('ref_axis',(1.,0.,0.));
#10308=DIRECTION('',(0.,0.,1.));
#10309=DIRECTION('center_axis',(0.,0.,-1.));
#10310=DIRECTION('ref_axis',(1.,0.,0.));
#10311=DIRECTION('center_axis',(0.,0.,1.));
#10312=DIRECTION('ref_axis',(1.,0.,0.));
#10313=DIRECTION('center_axis',(0.,0.,1.));
#10314=DIRECTION('ref_axis',(1.,0.,0.));
#10315=DIRECTION('',(0.,0.,1.));
#10316=DIRECTION('center_axis',(0.,0.,-1.));
#10317=DIRECTION('ref_axis',(1.,0.,0.));
#10318=DIRECTION('center_axis',(0.,0.,1.));
#10319=DIRECTION('ref_axis',(1.,0.,0.));
#10320=DIRECTION('center_axis',(0.,0.,1.));
#10321=DIRECTION('ref_axis',(1.,0.,0.));
#10322=DIRECTION('',(0.,0.,1.));
#10323=DIRECTION('center_axis',(0.,0.,-1.));
#10324=DIRECTION('ref_axis',(1.,0.,0.));
#10325=DIRECTION('center_axis',(0.,0.,1.));
#10326=DIRECTION('ref_axis',(1.,0.,0.));
#10327=DIRECTION('center_axis',(0.,0.,1.));
#10328=DIRECTION('ref_axis',(1.,0.,0.));
#10329=DIRECTION('',(0.,0.,1.));
#10330=DIRECTION('center_axis',(0.,0.,-1.));
#10331=DIRECTION('ref_axis',(1.,0.,0.));
#10332=DIRECTION('center_axis',(0.,0.,1.));
#10333=DIRECTION('ref_axis',(1.,0.,0.));
#10334=DIRECTION('center_axis',(0.,0.,1.));
#10335=DIRECTION('ref_axis',(1.,0.,0.));
#10336=DIRECTION('',(0.,0.,1.));
#10337=DIRECTION('center_axis',(0.,0.,-1.));
#10338=DIRECTION('ref_axis',(1.,0.,0.));
#10339=DIRECTION('center_axis',(0.,0.,1.));
#10340=DIRECTION('ref_axis',(1.,0.,0.));
#10341=DIRECTION('center_axis',(0.,0.,1.));
#10342=DIRECTION('ref_axis',(1.,0.,0.));
#10343=DIRECTION('',(0.,0.,1.));
#10344=DIRECTION('center_axis',(0.,0.,-1.));
#10345=DIRECTION('ref_axis',(1.,0.,0.));
#10346=DIRECTION('center_axis',(0.,1.,0.));
#10347=DIRECTION('ref_axis',(-1.,0.,0.));
#10348=DIRECTION('',(-1.,0.,0.));
#10349=DIRECTION('',(0.,0.,1.));
#10350=DIRECTION('',(-1.,0.,0.));
#10351=DIRECTION('',(0.,0.,1.));
#10352=DIRECTION('center_axis',(1.,0.,0.));
#10353=DIRECTION('ref_axis',(0.,1.,0.));
#10354=DIRECTION('',(0.,1.,0.));
#10355=DIRECTION('',(0.,1.,0.));
#10356=DIRECTION('',(0.,0.,1.));
#10357=DIRECTION('center_axis',(0.,-1.,0.));
#10358=DIRECTION('ref_axis',(1.,0.,0.));
#10359=DIRECTION('',(1.,0.,0.));
#10360=DIRECTION('',(1.,0.,0.));
#10361=DIRECTION('',(0.,0.,1.));
#10362=DIRECTION('center_axis',(-1.,0.,0.));
#10363=DIRECTION('ref_axis',(0.,-1.,0.));
#10364=DIRECTION('',(0.,-1.,0.));
#10365=DIRECTION('',(0.,-1.,0.));
#10366=DIRECTION('center_axis',(0.,0.,1.));
#10367=DIRECTION('ref_axis',(1.,0.,0.));
#10368=DIRECTION('center_axis',(0.,0.,1.));
#10369=DIRECTION('ref_axis',(1.,0.,0.));
#13005=CARTESIAN_POINT('',(0.,0.,0.));
#13006=CARTESIAN_POINT('Origin',(13.,-1.8,-0.1));
#13007=CARTESIAN_POINT('',(12.79,-1.8,0.));
#13008=CARTESIAN_POINT('Origin',(13.,-1.8,0.));
#13009=CARTESIAN_POINT('',(12.79,-1.8,1.));
#13010=CARTESIAN_POINT('',(12.79,-1.8,-0.1));
#13011=CARTESIAN_POINT('Origin',(13.,-1.8,1.));
#13012=CARTESIAN_POINT('Origin',(17.,1.8,-0.1));
#13013=CARTESIAN_POINT('',(16.79,1.8,0.));
#13014=CARTESIAN_POINT('Origin',(17.,1.8,0.));
#13015=CARTESIAN_POINT('',(16.79,1.8,1.));
#13016=CARTESIAN_POINT('',(16.79,1.8,-0.1));
#13017=CARTESIAN_POINT('Origin',(17.,1.8,1.));
#13018=CARTESIAN_POINT('Origin',(13.,1.8,-0.1));
#13019=CARTESIAN_POINT('',(12.79,1.8,0.));
#13020=CARTESIAN_POINT('Origin',(13.,1.8,0.));
#13021=CARTESIAN_POINT('',(12.79,1.8,1.));
#13022=CARTESIAN_POINT('',(12.79,1.8,-0.1));
#13023=CARTESIAN_POINT('Origin',(13.,1.8,1.));
#13024=CARTESIAN_POINT('Origin',(17.,-1.8,-0.1));
#13025=CARTESIAN_POINT('',(16.79,-1.8,0.));
#13026=CARTESIAN_POINT('Origin',(17.,-1.8,0.));
#13027=CARTESIAN_POINT('',(16.79,-1.8,1.));
#13028=CARTESIAN_POINT('',(16.79,-1.8,-0.1));
#13029=CARTESIAN_POINT('Origin',(17.,-1.8,1.));
#13030=CARTESIAN_POINT('Origin',(-1.8,-13.,-0.1));
#13031=CARTESIAN_POINT('',(-2.01,-13.,0.));
#13032=CARTESIAN_POINT('Origin',(-1.8,-13.,0.));
#13033=CARTESIAN_POINT('',(-2.01,-13.,1.));
#13034=CARTESIAN_POINT('',(-2.01,-13.,-0.1));
#13035=CARTESIAN_POINT('Origin',(-1.8,-13.,1.));
#13036=CARTESIAN_POINT('Origin',(1.8,-17.,-0.1));
#13037=CARTESIAN_POINT('',(1.59,-17.,0.));
#13038=CARTESIAN_POINT('Origin',(1.8,-17.,0.));
#13039=CARTESIAN_POINT('',(1.59,-17.,1.));
#13040=CARTESIAN_POINT('',(1.59,-17.,-0.1));
#13041=CARTESIAN_POINT('Origin',(1.8,-17.,1.));
#13042=CARTESIAN_POINT('Origin',(1.8,-13.,-0.1));
#13043=CARTESIAN_POINT('',(1.59,-13.,0.));
#13044=CARTESIAN_POINT('Origin',(1.8,-13.,0.));
#13045=CARTESIAN_POINT('',(1.59,-13.,1.));
#13046=CARTESIAN_POINT('',(1.59,-13.,-0.1));
#13047=CARTESIAN_POINT('Origin',(1.8,-13.,1.));
#13048=CARTESIAN_POINT('Origin',(-1.8,-17.,-0.1));
#13049=CARTESIAN_POINT('',(-2.01,-17.,0.));
#13050=CARTESIAN_POINT('Origin',(-1.8,-17.,0.));
#13051=CARTESIAN_POINT('',(-2.01,-17.,1.));
#13052=CARTESIAN_POINT('',(-2.01,-17.,-0.1));
#13053=CARTESIAN_POINT('Origin',(-1.8,-17.,1.));
#13054=CARTESIAN_POINT('Origin',(-13.,1.8,-0.1));
#13055=CARTESIAN_POINT('',(-13.21,1.8,0.));
#13056=CARTESIAN_POINT('Origin',(-13.,1.8,0.));
#13057=CARTESIAN_POINT('',(-13.21,1.8,1.));
#13058=CARTESIAN_POINT('',(-13.21,1.8,-0.1));
#13059=CARTESIAN_POINT('Origin',(-13.,1.8,1.));
#13060=CARTESIAN_POINT('Origin',(-17.,-1.8,-0.1));
#13061=CARTESIAN_POINT('',(-17.21,-1.8,0.));
#13062=CARTESIAN_POINT('Origin',(-17.,-1.8,0.));
#13063=CARTESIAN_POINT('',(-17.21,-1.8,1.));
#13064=CARTESIAN_POINT('',(-17.21,-1.8,-0.1));
#13065=CARTESIAN_POINT('Origin',(-17.,-1.8,1.));
#13066=CARTESIAN_POINT('Origin',(-13.,-1.8,-0.1));
#13067=CARTESIAN_POINT('',(-13.21,-1.8,0.));
#13068=CARTESIAN_POINT('Origin',(-13.,-1.8,0.));
#13069=CARTESIAN_POINT('',(-13.21,-1.8,1.));
#13070=CARTESIAN_POINT('',(-13.21,-1.8,-0.1));
#13071=CARTESIAN_POINT('Origin',(-13.,-1.8,1.));
#13072=CARTESIAN_POINT('Origin',(-17.,1.8,-0.1));
#13073=CARTESIAN_POINT('',(-17.21,1.8,0.));
#13074=CARTESIAN_POINT('Origin',(-17.,1.8,0.));
#13075=CARTESIAN_POINT('',(-17.21,1.8,1.));
#13076=CARTESIAN_POINT('',(-17.21,1.8,-0.1));
#13077=CARTESIAN_POINT('Origin',(-17.,1.8,1.));
#13078=CARTESIAN_POINT('Origin',(1.8,13.,-0.1));
#13079=CARTESIAN_POINT('',(1.59,13.,0.));
#13080=CARTESIAN_POINT('Origin',(1.8,13.,0.));
#13081=CARTESIAN_POINT('',(1.59,13.,1.));
#13082=CARTESIAN_POINT('',(1.59,13.,-0.1));
#13083=CARTESIAN_POINT('Origin',(1.8,13.,1.));
#13084=CARTESIAN_POINT('Origin',(-1.8,17.,-0.1));
#13085=CARTESIAN_POINT('',(-2.01,17.,0.));
#13086=CARTESIAN_POINT('Origin',(-1.8,17.,0.));
#13087=CARTESIAN_POINT('',(-2.01,17.,1.));
#13088=CARTESIAN_POINT('',(-2.01,17.,-0.1));
#13089=CARTESIAN_POINT('Origin',(-1.8,17.,1.));
#13090=CARTESIAN_POINT('Origin',(-1.8,13.,-0.1));
#13091=CARTESIAN_POINT('',(-2.01,13.,0.));
#13092=CARTESIAN_POINT('Origin',(-1.8,13.,0.));
#13093=CARTESIAN_POINT('',(-2.01,13.,1.));
#13094=CARTESIAN_POINT('',(-2.01,13.,-0.1));
#13095=CARTESIAN_POINT('Origin',(-1.8,13.,1.));
#13096=CARTESIAN_POINT('Origin',(1.8,17.,-0.1));
#13097=CARTESIAN_POINT('',(1.59,17.,0.));
#13098=CARTESIAN_POINT('Origin',(1.8,17.,0.));
#13099=CARTESIAN_POINT('',(1.59,17.,1.));
#13100=CARTESIAN_POINT('',(1.59,17.,-0.1));
#13101=CARTESIAN_POINT('Origin',(1.8,17.,1.));
#13102=CARTESIAN_POINT('Origin',(-2.40416305603426,-2.40416305603426,-0.1));
#13103=CARTESIAN_POINT('',(-2.65416305603426,-2.40416305603426,0.));
#13104=CARTESIAN_POINT('Origin',(-2.40416305603426,-2.40416305603426,0.));
#13105=CARTESIAN_POINT('',(-2.65416305603426,-2.40416305603426,1.));
#13106=CARTESIAN_POINT('',(-2.65416305603426,-2.40416305603426,-0.1));
#13107=CARTESIAN_POINT('Origin',(-2.40416305603426,-2.40416305603426,1.));
#13108=CARTESIAN_POINT('Origin',(-2.40416305603426,2.40416305603426,-0.1));
#13109=CARTESIAN_POINT('',(-2.65416305603426,2.40416305603426,0.));
#13110=CARTESIAN_POINT('Origin',(-2.40416305603426,2.40416305603426,0.));
#13111=CARTESIAN_POINT('',(-2.65416305603426,2.40416305603426,1.));
#13112=CARTESIAN_POINT('',(-2.65416305603426,2.40416305603426,-0.1));
#13113=CARTESIAN_POINT('Origin',(-2.40416305603426,2.40416305603426,1.));
#13114=CARTESIAN_POINT('Origin',(2.40416305603426,2.40416305603426,-0.1));
#13115=CARTESIAN_POINT('',(2.15416305603426,2.40416305603426,0.));
#13116=CARTESIAN_POINT('Origin',(2.40416305603426,2.40416305603426,0.));
#13117=CARTESIAN_POINT('',(2.15416305603426,2.40416305603426,1.));
#13118=CARTESIAN_POINT('',(2.15416305603426,2.40416305603426,-0.1));
#13119=CARTESIAN_POINT('Origin',(2.40416305603426,2.40416305603426,1.));
#13120=CARTESIAN_POINT('Origin',(2.40416305603426,-2.40416305603426,-0.1));
#13121=CARTESIAN_POINT('',(2.15416305603426,-2.40416305603426,0.));
#13122=CARTESIAN_POINT('Origin',(2.40416305603426,-2.40416305603426,0.));
#13123=CARTESIAN_POINT('',(2.15416305603426,-2.40416305603426,1.));
#13124=CARTESIAN_POINT('',(2.15416305603426,-2.40416305603426,-0.1));
#13125=CARTESIAN_POINT('Origin',(2.40416305603426,-2.40416305603426,1.));
#13126=CARTESIAN_POINT('Origin',(21.,21.,0.));
#13127=CARTESIAN_POINT('',(21.,21.,0.));
#13128=CARTESIAN_POINT('',(-21.,21.,0.));
#13129=CARTESIAN_POINT('',(21.,21.,0.));
#13130=CARTESIAN_POINT('',(-21.,21.,1.));
#13131=CARTESIAN_POINT('',(-21.,21.,0.));
#13132=CARTESIAN_POINT('',(21.,21.,1.));
#13133=CARTESIAN_POINT('',(21.,21.,1.));
#13134=CARTESIAN_POINT('',(21.,21.,0.));
#13135=CARTESIAN_POINT('Origin',(21.,-21.,0.));
#13136=CARTESIAN_POINT('',(21.,-21.,0.));
#13137=CARTESIAN_POINT('',(21.,-21.,0.));
#13138=CARTESIAN_POINT('',(21.,-21.,1.));
#13139=CARTESIAN_POINT('',(21.,-21.,1.));
#13140=CARTESIAN_POINT('',(21.,-21.,0.));
#13141=CARTESIAN_POINT('Origin',(-21.,-21.,0.));
#13142=CARTESIAN_POINT('',(-21.,-21.,0.));
#13143=CARTESIAN_POINT('',(-21.,-21.,0.));
#13144=CARTESIAN_POINT('',(-21.,-21.,1.));
#13145=CARTESIAN_POINT('',(-21.,-21.,1.));
#13146=CARTESIAN_POINT('',(-21.,-21.,0.));
#13147=CARTESIAN_POINT('Origin',(-21.,21.,0.));
#13148=CARTESIAN_POINT('',(-21.,21.,0.));
#13149=CARTESIAN_POINT('',(-21.,21.,1.));
#13150=CARTESIAN_POINT('Origin',(0.,0.,1.));
#13151=CARTESIAN_POINT('Origin',(0.,0.,0.));
#16146=UNCERTAINTY_MEASURE_WITH_UNIT(LENGTH_MEASURE(0.001),#16282,
'DISTANCE_ACCURACY_VALUE',
'Maximum model space distance between geometric entities at asserted c
onnectivities');
#16212=UNCERTAINTY_MEASURE_WITH_UNIT(LENGTH_MEASURE(0.001),#16282,
'DISTANCE_ACCURACY_VALUE',
'Maximum model space distance between geometric entities at asserted c
onnectivities');
#16215=(
GEOMETRIC_REPRESENTATION_CONTEXT(3)
GLOBAL_UNCERTAINTY_ASSIGNED_CONTEXT((#16146))
GLOBAL_UNIT_ASSIGNED_CONTEXT((#16282,#16284,#16285))
REPRESENTATION_CONTEXT('','3D')
);
#16281=(
GEOMETRIC_REPRESENTATION_CONTEXT(3)
GLOBAL_UNCERTAINTY_ASSIGNED_CONTEXT((#16212))
GLOBAL_UNIT_ASSIGNED_CONTEXT((#16282,#16284,#16285))
REPRESENTATION_CONTEXT('','3D')
);
#16282=(
LENGTH_UNIT()
NAMED_UNIT(*)
SI_UNIT(.CENTI.,.METRE.)
);
#16284=(
NAMED_UNIT(*)
PLANE_ANGLE_UNIT()
SI_UNIT($,.RADIAN.)
);
#16285=(
NAMED_UNIT(*)
SI_UNIT($,.STERADIAN.)
SOLID_ANGLE_UNIT()
);
#16288=SHAPE_DEFINITION_REPRESENTATION(#16356,#16521);
#16356=PRODUCT_DEFINITION_SHAPE('',$,#16590);
#16521=SHAPE_REPRESENTATION('',(#9042),#16215);
#16587=PRODUCT_DEFINITION_CONTEXT('part definition',#16793,'design');
#16590=PRODUCT_DEFINITION('Base','Base',#16658,#16587);
#16658=PRODUCT_DEFINITION_FORMATION('',$,#16797);
#16793=APPLICATION_CONTEXT(
'Core Data for Automotive Mechanical Design Process');
#16794=PRODUCT_CONTEXT('part definition',#16793,'mechanical');
#16797=PRODUCT('Base','Base','Base',(#16794));
#16905=COLOUR_RGB('Dark Blue',0.08,0.2,0.34);
#16906=FILL_AREA_STYLE_COLOUR('',#16905);
#16907=FILL_AREA_STYLE('',(#16906));
#16908=SURFACE_STYLE_FILL_AREA(#16907);
#16909=SURFACE_SIDE_STYLE('',(#16908));
#16910=SURFACE_STYLE_USAGE(.BOTH.,#16909);
#16911=PRESENTATION_STYLE_ASSIGNMENT((#16910));
ENDSEC;
END-ISO-10303-21;
